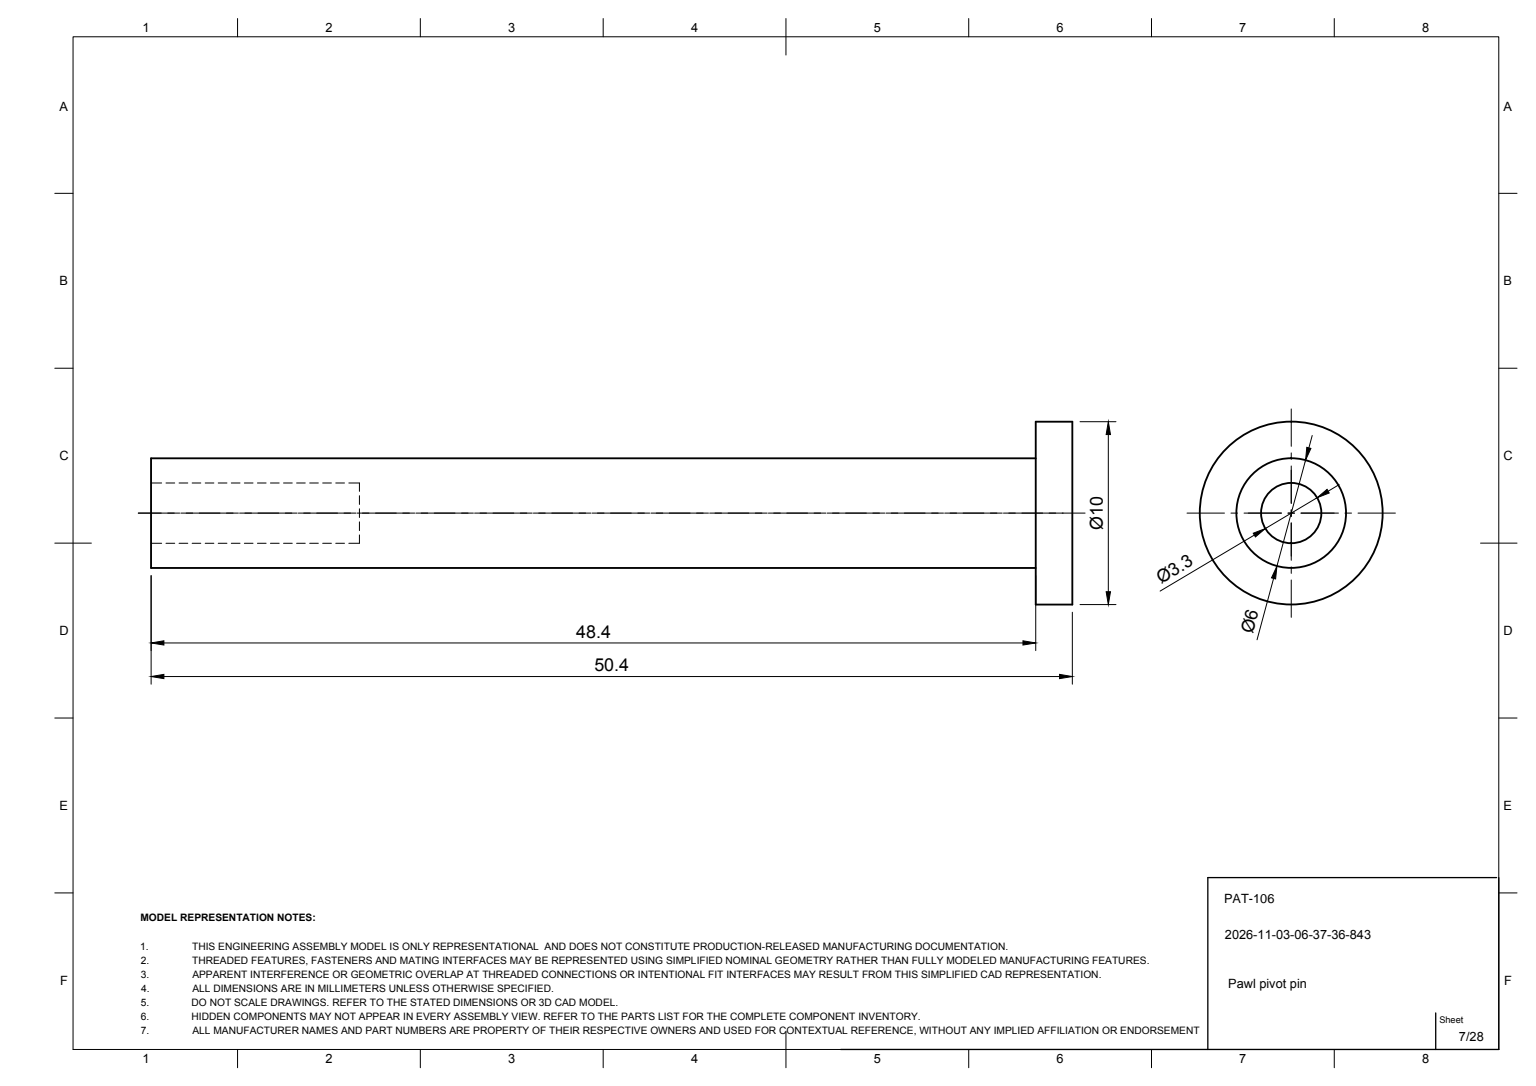
ISO-10303-21;
HEADER;
/* Generated by software containing ST-Developer
 * from STEP Tools, Inc. (www.steptools.com) 
 */

FILE_DESCRIPTION(
/* description */ ('Torsion-spring ratchet demonstrator'),
/* implementation_level */ '2;1');

FILE_NAME(
/* name */ 'Pawl pivot pin.step',
/* time_stamp */ '2026-10-29T17:29:17-07:00',
/* author */ (''),
/* organization */ (''),
/* preprocessor_version */ 'ST-DEVELOPER v20.2',
/* originating_system */ 'Autodesk Translation Framework v15.17.0.0',
/* authorisation */ '');

FILE_SCHEMA (('AUTOMOTIVE_DESIGN { 1 0 10303 214 3 1 1 }'));
ENDSEC;

DATA;
#10=MECHANICAL_DESIGN_GEOMETRIC_PRESENTATION_REPRESENTATION('',(#285),#11258);
#237=SHAPE_REPRESENTATION_RELATIONSHIP('SRR','None',#11363,#261);
#261=ADVANCED_BREP_SHAPE_REPRESENTATION('',(#317),#11233);
#285=STYLED_ITEM('',(#11584),#317);
#317=MANIFOLD_SOLID_BREP('Body1',#5156);
#367=FACE_BOUND('',#979,.T.);
#368=FACE_BOUND('',#984,.T.);
#451=PLANE('',#5511);
#452=PLANE('',#5512);
#453=PLANE('',#5517);
#454=PLANE('',#5520);
#649=FACE_OUTER_BOUND('',#976,.T.);
#650=FACE_OUTER_BOUND('',#977,.T.);
#651=FACE_OUTER_BOUND('',#978,.T.);
#652=FACE_OUTER_BOUND('',#980,.T.);
#653=FACE_OUTER_BOUND('',#981,.T.);
#654=FACE_OUTER_BOUND('',#982,.T.);
#655=FACE_OUTER_BOUND('',#983,.T.);
#976=EDGE_LOOP('',(#3562,#3563,#3564,#3565));
#977=EDGE_LOOP('',(#3566));
#978=EDGE_LOOP('',(#3567));
#979=EDGE_LOOP('',(#3568));
#980=EDGE_LOOP('',(#3569,#3570,#3571,#3572));
#981=EDGE_LOOP('',(#3573));
#982=EDGE_LOOP('',(#3574,#3575,#3576,#3577));
#983=EDGE_LOOP('',(#3578));
#984=EDGE_LOOP('',(#3579));
#1361=LINE('',#7810,#1744);
#1362=LINE('',#7820,#1745);
#1363=LINE('',#7826,#1746);
#1744=VECTOR('',#6216,0.165);
#1745=VECTOR('',#6229,0.5);
#1746=VECTOR('',#6238,0.3);
#2115=CIRCLE('',#5509,0.165);
#2116=CIRCLE('',#5510,0.165);
#2117=CIRCLE('',#5513,0.5);
#2118=CIRCLE('',#5514,0.3);
#2119=CIRCLE('',#5516,0.5);
#2120=CIRCLE('',#5519,0.3);
#2375=VERTEX_POINT('',#7807);
#2376=VERTEX_POINT('',#7809);
#2377=VERTEX_POINT('',#7814);
#2378=VERTEX_POINT('',#7816);
#2379=VERTEX_POINT('',#7819);
#2380=VERTEX_POINT('',#7824);
#2841=EDGE_CURVE('',#2375,#2375,#2115,.T.);
#2842=EDGE_CURVE('',#2375,#2376,#1361,.T.);
#2843=EDGE_CURVE('',#2376,#2376,#2116,.T.);
#2844=EDGE_CURVE('',#2377,#2377,#2117,.T.);
#2845=EDGE_CURVE('',#2378,#2378,#2118,.T.);
#2846=EDGE_CURVE('',#2377,#2379,#1362,.T.);
#2847=EDGE_CURVE('',#2379,#2379,#2119,.T.);
#2848=EDGE_CURVE('',#2380,#2380,#2120,.T.);
#2849=EDGE_CURVE('',#2380,#2378,#1363,.T.);
#3562=ORIENTED_EDGE('',*,*,#2841,.F.);
#3563=ORIENTED_EDGE('',*,*,#2842,.T.);
#3564=ORIENTED_EDGE('',*,*,#2843,.F.);
#3565=ORIENTED_EDGE('',*,*,#2842,.F.);
#3566=ORIENTED_EDGE('',*,*,#2841,.T.);
#3567=ORIENTED_EDGE('',*,*,#2844,.T.);
#3568=ORIENTED_EDGE('',*,*,#2845,.F.);
#3569=ORIENTED_EDGE('',*,*,#2844,.F.);
#3570=ORIENTED_EDGE('',*,*,#2846,.T.);
#3571=ORIENTED_EDGE('',*,*,#2847,.T.);
#3572=ORIENTED_EDGE('',*,*,#2846,.F.);
#3573=ORIENTED_EDGE('',*,*,#2847,.F.);
#3574=ORIENTED_EDGE('',*,*,#2848,.F.);
#3575=ORIENTED_EDGE('',*,*,#2849,.T.);
#3576=ORIENTED_EDGE('',*,*,#2845,.T.);
#3577=ORIENTED_EDGE('',*,*,#2849,.F.);
#3578=ORIENTED_EDGE('',*,*,#2848,.T.);
#3579=ORIENTED_EDGE('',*,*,#2843,.T.);
#4776=CYLINDRICAL_SURFACE('',#5508,0.165);
#4777=CYLINDRICAL_SURFACE('',#5515,0.5);
#4778=CYLINDRICAL_SURFACE('',#5518,0.3);
#4875=ADVANCED_FACE('',(#649),#4776,.F.);
#4876=ADVANCED_FACE('',(#650),#451,.T.);
#4877=ADVANCED_FACE('',(#651,#367),#452,.T.);
#4878=ADVANCED_FACE('',(#652),#4777,.T.);
#4879=ADVANCED_FACE('',(#653),#453,.F.);
#4880=ADVANCED_FACE('',(#654),#4778,.T.);
#4881=ADVANCED_FACE('',(#655,#368),#454,.T.);
#5156=CLOSED_SHELL('',(#4875,#4876,#4877,#4878,#4879,#4880,#4881));
#5507=AXIS2_PLACEMENT_3D('',#7805,#6210,#6211);
#5508=AXIS2_PLACEMENT_3D('',#7806,#6212,#6213);
#5509=AXIS2_PLACEMENT_3D('',#7808,#6214,#6215);
#5510=AXIS2_PLACEMENT_3D('',#7811,#6217,#6218);
#5511=AXIS2_PLACEMENT_3D('',#7812,#6219,#6220);
#5512=AXIS2_PLACEMENT_3D('',#7813,#6221,#6222);
#5513=AXIS2_PLACEMENT_3D('',#7815,#6223,#6224);
#5514=AXIS2_PLACEMENT_3D('',#7817,#6225,#6226);
#5515=AXIS2_PLACEMENT_3D('',#7818,#6227,#6228);
#5516=AXIS2_PLACEMENT_3D('',#7821,#6230,#6231);
#5517=AXIS2_PLACEMENT_3D('',#7822,#6232,#6233);
#5518=AXIS2_PLACEMENT_3D('',#7823,#6234,#6235);
#5519=AXIS2_PLACEMENT_3D('',#7825,#6236,#6237);
#5520=AXIS2_PLACEMENT_3D('',#7827,#6239,#6240);
#6210=DIRECTION('axis',(0.,0.,1.));
#6211=DIRECTION('refdir',(1.,0.,0.));
#6212=DIRECTION('center_axis',(0.,0.,1.));
#6213=DIRECTION('ref_axis',(1.,0.,0.));
#6214=DIRECTION('center_axis',(0.,0.,1.));
#6215=DIRECTION('ref_axis',(1.,0.,0.));
#6216=DIRECTION('',(0.,0.,1.));
#6217=DIRECTION('center_axis',(0.,0.,-1.));
#6218=DIRECTION('ref_axis',(1.,0.,0.));
#6219=DIRECTION('center_axis',(0.,0.,1.));
#6220=DIRECTION('ref_axis',(1.,0.,0.));
#6221=DIRECTION('center_axis',(0.,0.,1.));
#6222=DIRECTION('ref_axis',(1.,0.,0.));
#6223=DIRECTION('center_axis',(0.,0.,1.));
#6224=DIRECTION('ref_axis',(1.,0.,0.));
#6225=DIRECTION('center_axis',(0.,0.,1.));
#6226=DIRECTION('ref_axis',(1.,0.,0.));
#6227=DIRECTION('center_axis',(0.,0.,1.));
#6228=DIRECTION('ref_axis',(1.,0.,0.));
#6229=DIRECTION('',(0.,0.,-1.));
#6230=DIRECTION('center_axis',(0.,0.,1.));
#6231=DIRECTION('ref_axis',(1.,0.,0.));
#6232=DIRECTION('center_axis',(0.,0.,1.));
#6233=DIRECTION('ref_axis',(1.,0.,0.));
#6234=DIRECTION('center_axis',(0.,0.,1.));
#6235=DIRECTION('ref_axis',(1.,0.,0.));
#6236=DIRECTION('center_axis',(0.,0.,1.));
#6237=DIRECTION('ref_axis',(1.,0.,0.));
#6238=DIRECTION('',(0.,0.,-1.));
#6239=DIRECTION('center_axis',(0.,0.,1.));
#6240=DIRECTION('ref_axis',(1.,0.,0.));
#7805=CARTESIAN_POINT('',(0.,0.,0.));
#7806=CARTESIAN_POINT('Origin',(6.5,-3.47,5.5));
#7807=CARTESIAN_POINT('',(6.335,-3.47,5.5));
#7808=CARTESIAN_POINT('Origin',(6.5,-3.47,5.5));
#7809=CARTESIAN_POINT('',(6.335,-3.47,6.64));
#7810=CARTESIAN_POINT('',(6.335,-3.47,5.5));
#7811=CARTESIAN_POINT('Origin',(6.5,-3.47,6.64));
#7812=CARTESIAN_POINT('Origin',(6.5,-3.47,5.5));
#7813=CARTESIAN_POINT('Origin',(6.5,-3.47,1.8));
#7814=CARTESIAN_POINT('',(6.,-3.47,1.8));
#7815=CARTESIAN_POINT('Origin',(6.5,-3.47,1.8));
#7816=CARTESIAN_POINT('',(6.2,-3.47,1.8));
#7817=CARTESIAN_POINT('Origin',(6.5,-3.47,1.8));
#7818=CARTESIAN_POINT('Origin',(6.5,-3.47,1.6));
#7819=CARTESIAN_POINT('',(6.,-3.47,1.6));
#7820=CARTESIAN_POINT('',(6.,-3.47,1.6));
#7821=CARTESIAN_POINT('Origin',(6.5,-3.47,1.6));
#7822=CARTESIAN_POINT('Origin',(6.5,-3.47,1.6));
#7823=CARTESIAN_POINT('Origin',(6.5,-3.47,1.8));
#7824=CARTESIAN_POINT('',(6.2,-3.47,6.64));
#7825=CARTESIAN_POINT('Origin',(6.5,-3.47,6.64));
#7826=CARTESIAN_POINT('',(6.2,-3.47,1.8));
#7827=CARTESIAN_POINT('Origin',(6.5,-3.47,6.64));
#11203=UNCERTAINTY_MEASURE_WITH_UNIT(LENGTH_MEASURE(0.001),#11259,
'DISTANCE_ACCURACY_VALUE',
'Maximum model space distance between geometric entities at asserted c
onnectivities');
#11228=UNCERTAINTY_MEASURE_WITH_UNIT(LENGTH_MEASURE(0.001),#11259,
'DISTANCE_ACCURACY_VALUE',
'Maximum model space distance between geometric entities at asserted c
onnectivities');
#11233=(
GEOMETRIC_REPRESENTATION_CONTEXT(3)
GLOBAL_UNCERTAINTY_ASSIGNED_CONTEXT((#11203))
GLOBAL_UNIT_ASSIGNED_CONTEXT((#11259,#11261,#11262))
REPRESENTATION_CONTEXT('','3D')
);
#11258=(
GEOMETRIC_REPRESENTATION_CONTEXT(3)
GLOBAL_UNCERTAINTY_ASSIGNED_CONTEXT((#11228))
GLOBAL_UNIT_ASSIGNED_CONTEXT((#11259,#11261,#11262))
REPRESENTATION_CONTEXT('','3D')
);
#11259=(
LENGTH_UNIT()
NAMED_UNIT(*)
SI_UNIT(.CENTI.,.METRE.)
);
#11261=(
NAMED_UNIT(*)
PLANE_ANGLE_UNIT()
SI_UNIT($,.RADIAN.)
);
#11262=(
NAMED_UNIT(*)
SI_UNIT($,.STERADIAN.)
SOLID_ANGLE_UNIT()
);
#11267=SHAPE_DEFINITION_REPRESENTATION(#11296,#11363);
#11296=PRODUCT_DEFINITION_SHAPE('',$,#11393);
#11363=SHAPE_REPRESENTATION('',(#5507),#11233);
#11388=PRODUCT_DEFINITION_CONTEXT('part definition',#11477,'design');
#11393=PRODUCT_DEFINITION('Pawl pivot pin','Pawl pivot pin',#11422,#11388);
#11422=PRODUCT_DEFINITION_FORMATION('',$,#11483);
#11477=APPLICATION_CONTEXT(
'Core Data for Automotive Mechanical Design Process');
#11478=PRODUCT_CONTEXT('part definition',#11477,'mechanical');
#11483=PRODUCT('Pawl pivot pin','Pawl pivot pin','Pawl pivot pin',(#11478));
#11578=COLOUR_RGB('Grey',0.48,0.52,0.57);
#11579=FILL_AREA_STYLE_COLOUR('',#11578);
#11580=FILL_AREA_STYLE('',(#11579));
#11581=SURFACE_STYLE_FILL_AREA(#11580);
#11582=SURFACE_SIDE_STYLE('',(#11581));
#11583=SURFACE_STYLE_USAGE(.BOTH.,#11582);
#11584=PRESENTATION_STYLE_ASSIGNMENT((#11583));
ENDSEC;
END-ISO-10303-21;
